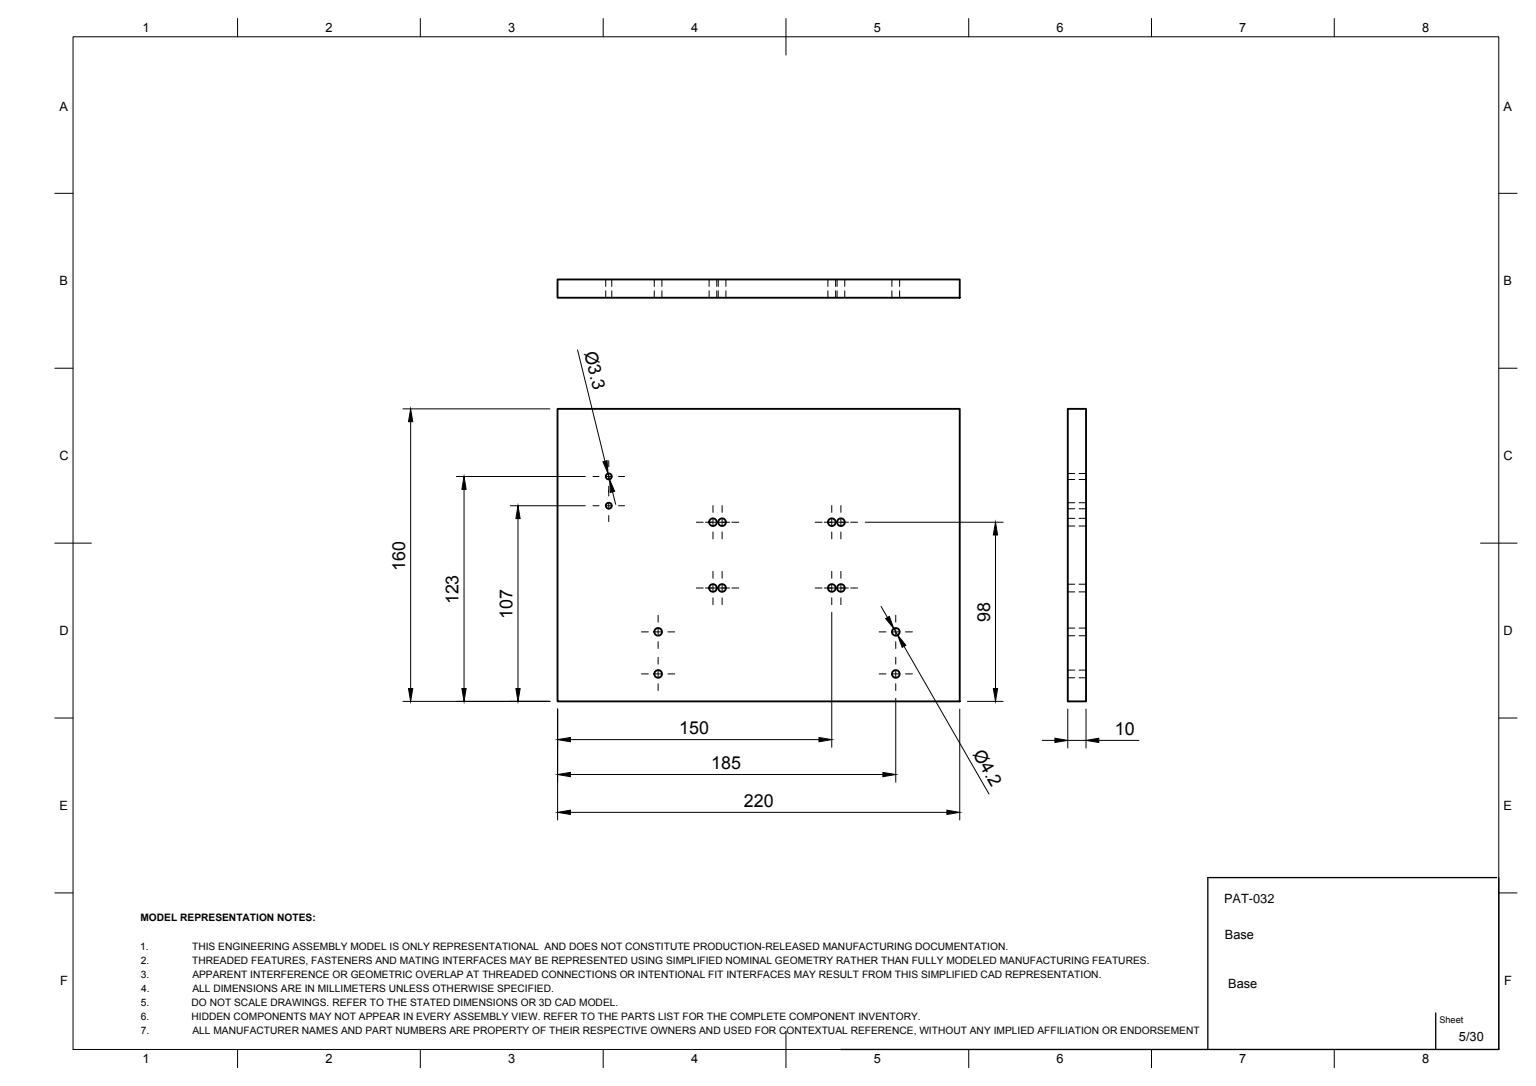
ISO-10303-21;
HEADER;
/* Generated by software containing ST-Developer
 * from STEP Tools, Inc. (www.steptools.com) 
 */

FILE_DESCRIPTION(
/* description */ ('Drill jig with bushing plate'),
/* implementation_level */ '2;1');

FILE_NAME(
/* name */ 'Base.step',
/* time_stamp */ '2026-10-27T10:51:08-07:00',
/* author */ (''),
/* organization */ (''),
/* preprocessor_version */ 'ST-DEVELOPER v20.2',
/* originating_system */ 'Autodesk Translation Framework v15.17.0.0',
/* authorisation */ '');

FILE_SCHEMA (('AUTOMOTIVE_DESIGN { 1 0 10303 214 3 1 1 }'));
ENDSEC;

DATA;
#10=MECHANICAL_DESIGN_GEOMETRIC_PRESENTATION_REPRESENTATION('',(#223),#6638);
#175=SHAPE_REPRESENTATION_RELATIONSHIP('SRR','None',#6739,#199);
#199=ADVANCED_BREP_SHAPE_REPRESENTATION('',(#247),#6612);
#223=STYLED_ITEM('',(#6922),#247);
#247=MANIFOLD_SOLID_BREP('Body1',#3590);
#269=FACE_BOUND('',#734,.T.);
#270=FACE_BOUND('',#735,.T.);
#271=FACE_BOUND('',#736,.T.);
#272=FACE_BOUND('',#737,.T.);
#273=FACE_BOUND('',#738,.T.);
#274=FACE_BOUND('',#739,.T.);
#275=FACE_BOUND('',#740,.T.);
#276=FACE_BOUND('',#741,.T.);
#277=FACE_BOUND('',#742,.T.);
#278=FACE_BOUND('',#743,.T.);
#279=FACE_BOUND('',#744,.T.);
#280=FACE_BOUND('',#745,.T.);
#281=FACE_BOUND('',#746,.T.);
#282=FACE_BOUND('',#747,.T.);
#283=FACE_BOUND('',#749,.T.);
#284=FACE_BOUND('',#750,.T.);
#285=FACE_BOUND('',#751,.T.);
#286=FACE_BOUND('',#752,.T.);
#287=FACE_BOUND('',#753,.T.);
#288=FACE_BOUND('',#754,.T.);
#289=FACE_BOUND('',#755,.T.);
#290=FACE_BOUND('',#756,.T.);
#291=FACE_BOUND('',#757,.T.);
#292=FACE_BOUND('',#758,.T.);
#293=FACE_BOUND('',#759,.T.);
#294=FACE_BOUND('',#760,.T.);
#295=FACE_BOUND('',#761,.T.);
#296=FACE_BOUND('',#762,.T.);
#370=PLANE('',#3926);
#371=PLANE('',#3927);
#372=PLANE('',#3928);
#373=PLANE('',#3929);
#374=PLANE('',#3930);
#375=PLANE('',#3931);
#501=FACE_OUTER_BOUND('',#715,.T.);
#502=FACE_OUTER_BOUND('',#716,.T.);
#503=FACE_OUTER_BOUND('',#717,.T.);
#504=FACE_OUTER_BOUND('',#718,.T.);
#505=FACE_OUTER_BOUND('',#719,.T.);
#506=FACE_OUTER_BOUND('',#720,.T.);
#507=FACE_OUTER_BOUND('',#721,.T.);
#508=FACE_OUTER_BOUND('',#722,.T.);
#509=FACE_OUTER_BOUND('',#723,.T.);
#510=FACE_OUTER_BOUND('',#724,.T.);
#511=FACE_OUTER_BOUND('',#725,.T.);
#512=FACE_OUTER_BOUND('',#726,.T.);
#513=FACE_OUTER_BOUND('',#727,.T.);
#514=FACE_OUTER_BOUND('',#728,.T.);
#515=FACE_OUTER_BOUND('',#729,.T.);
#516=FACE_OUTER_BOUND('',#730,.T.);
#517=FACE_OUTER_BOUND('',#731,.T.);
#518=FACE_OUTER_BOUND('',#732,.T.);
#519=FACE_OUTER_BOUND('',#733,.T.);
#520=FACE_OUTER_BOUND('',#748,.T.);
#715=EDGE_LOOP('',(#2437,#2438,#2439,#2440));
#716=EDGE_LOOP('',(#2441,#2442,#2443,#2444));
#717=EDGE_LOOP('',(#2445,#2446,#2447,#2448));
#718=EDGE_LOOP('',(#2449,#2450,#2451,#2452));
#719=EDGE_LOOP('',(#2453,#2454,#2455,#2456));
#720=EDGE_LOOP('',(#2457,#2458,#2459,#2460));
#721=EDGE_LOOP('',(#2461,#2462,#2463,#2464));
#722=EDGE_LOOP('',(#2465,#2466,#2467,#2468));
#723=EDGE_LOOP('',(#2469,#2470,#2471,#2472));
#724=EDGE_LOOP('',(#2473,#2474,#2475,#2476));
#725=EDGE_LOOP('',(#2477,#2478,#2479,#2480));
#726=EDGE_LOOP('',(#2481,#2482,#2483,#2484));
#727=EDGE_LOOP('',(#2485,#2486,#2487,#2488));
#728=EDGE_LOOP('',(#2489,#2490,#2491,#2492));
#729=EDGE_LOOP('',(#2493,#2494,#2495,#2496));
#730=EDGE_LOOP('',(#2497,#2498,#2499,#2500));
#731=EDGE_LOOP('',(#2501,#2502,#2503,#2504));
#732=EDGE_LOOP('',(#2505,#2506,#2507,#2508));
#733=EDGE_LOOP('',(#2509,#2510,#2511,#2512));
#734=EDGE_LOOP('',(#2513));
#735=EDGE_LOOP('',(#2514));
#736=EDGE_LOOP('',(#2515));
#737=EDGE_LOOP('',(#2516));
#738=EDGE_LOOP('',(#2517));
#739=EDGE_LOOP('',(#2518));
#740=EDGE_LOOP('',(#2519));
#741=EDGE_LOOP('',(#2520));
#742=EDGE_LOOP('',(#2521));
#743=EDGE_LOOP('',(#2522));
#744=EDGE_LOOP('',(#2523));
#745=EDGE_LOOP('',(#2524));
#746=EDGE_LOOP('',(#2525));
#747=EDGE_LOOP('',(#2526));
#748=EDGE_LOOP('',(#2527,#2528,#2529,#2530));
#749=EDGE_LOOP('',(#2531));
#750=EDGE_LOOP('',(#2532));
#751=EDGE_LOOP('',(#2533));
#752=EDGE_LOOP('',(#2534));
#753=EDGE_LOOP('',(#2535));
#754=EDGE_LOOP('',(#2536));
#755=EDGE_LOOP('',(#2537));
#756=EDGE_LOOP('',(#2538));
#757=EDGE_LOOP('',(#2539));
#758=EDGE_LOOP('',(#2540));
#759=EDGE_LOOP('',(#2541));
#760=EDGE_LOOP('',(#2542));
#761=EDGE_LOOP('',(#2543));
#762=EDGE_LOOP('',(#2544));
#1030=LINE('',#5493,#1291);
#1031=LINE('',#5499,#1292);
#1032=LINE('',#5505,#1293);
#1033=LINE('',#5511,#1294);
#1034=LINE('',#5517,#1295);
#1035=LINE('',#5523,#1296);
#1036=LINE('',#5529,#1297);
#1037=LINE('',#5535,#1298);
#1038=LINE('',#5541,#1299);
#1039=LINE('',#5547,#1300);
#1040=LINE('',#5553,#1301);
#1041=LINE('',#5559,#1302);
#1042=LINE('',#5565,#1303);
#1043=LINE('',#5571,#1304);
#1044=LINE('',#5576,#1305);
#1045=LINE('',#5578,#1306);
#1046=LINE('',#5580,#1307);
#1047=LINE('',#5581,#1308);
#1048=LINE('',#5584,#1309);
#1049=LINE('',#5586,#1310);
#1050=LINE('',#5587,#1311);
#1051=LINE('',#5590,#1312);
#1052=LINE('',#5592,#1313);
#1053=LINE('',#5593,#1314);
#1054=LINE('',#5595,#1315);
#1055=LINE('',#5596,#1316);
#1291=VECTOR('',#4339,0.164999999999999);
#1292=VECTOR('',#4346,0.164999999999999);
#1293=VECTOR('',#4353,0.21);
#1294=VECTOR('',#4360,0.21);
#1295=VECTOR('',#4367,0.21);
#1296=VECTOR('',#4374,0.21);
#1297=VECTOR('',#4381,0.21);
#1298=VECTOR('',#4388,0.21);
#1299=VECTOR('',#4395,0.21);
#1300=VECTOR('',#4402,0.21);
#1301=VECTOR('',#4409,0.21);
#1302=VECTOR('',#4416,0.21);
#1303=VECTOR('',#4423,0.21);
#1304=VECTOR('',#4430,0.21);
#1305=VECTOR('',#4435,1.);
#1306=VECTOR('',#4436,1.);
#1307=VECTOR('',#4437,1.);
#1308=VECTOR('',#4438,1.);
#1309=VECTOR('',#4441,1.);
#1310=VECTOR('',#4442,1.);
#1311=VECTOR('',#4443,1.);
#1312=VECTOR('',#4446,1.);
#1313=VECTOR('',#4447,1.);
#1314=VECTOR('',#4448,1.);
#1315=VECTOR('',#4451,1.);
#1316=VECTOR('',#4452,1.);
#1552=CIRCLE('',#3885,0.164999999999999);
#1553=CIRCLE('',#3886,0.164999999999999);
#1554=CIRCLE('',#3888,0.164999999999999);
#1555=CIRCLE('',#3889,0.164999999999999);
#1556=CIRCLE('',#3891,0.21);
#1557=CIRCLE('',#3892,0.21);
#1558=CIRCLE('',#3894,0.21);
#1559=CIRCLE('',#3895,0.21);
#1560=CIRCLE('',#3897,0.21);
#1561=CIRCLE('',#3898,0.21);
#1562=CIRCLE('',#3900,0.21);
#1563=CIRCLE('',#3901,0.21);
#1564=CIRCLE('',#3903,0.21);
#1565=CIRCLE('',#3904,0.21);
#1566=CIRCLE('',#3906,0.21);
#1567=CIRCLE('',#3907,0.21);
#1568=CIRCLE('',#3909,0.21);
#1569=CIRCLE('',#3910,0.21);
#1570=CIRCLE('',#3912,0.21);
#1571=CIRCLE('',#3913,0.21);
#1572=CIRCLE('',#3915,0.21);
#1573=CIRCLE('',#3916,0.21);
#1574=CIRCLE('',#3918,0.21);
#1575=CIRCLE('',#3919,0.21);
#1576=CIRCLE('',#3921,0.21);
#1577=CIRCLE('',#3922,0.21);
#1578=CIRCLE('',#3924,0.21);
#1579=CIRCLE('',#3925,0.21);
#1720=VERTEX_POINT('',#5490);
#1721=VERTEX_POINT('',#5492);
#1722=VERTEX_POINT('',#5496);
#1723=VERTEX_POINT('',#5498);
#1724=VERTEX_POINT('',#5502);
#1725=VERTEX_POINT('',#5504);
#1726=VERTEX_POINT('',#5508);
#1727=VERTEX_POINT('',#5510);
#1728=VERTEX_POINT('',#5514);
#1729=VERTEX_POINT('',#5516);
#1730=VERTEX_POINT('',#5520);
#1731=VERTEX_POINT('',#5522);
#1732=VERTEX_POINT('',#5526);
#1733=VERTEX_POINT('',#5528);
#1734=VERTEX_POINT('',#5532);
#1735=VERTEX_POINT('',#5534);
#1736=VERTEX_POINT('',#5538);
#1737=VERTEX_POINT('',#5540);
#1738=VERTEX_POINT('',#5544);
#1739=VERTEX_POINT('',#5546);
#1740=VERTEX_POINT('',#5550);
#1741=VERTEX_POINT('',#5552);
#1742=VERTEX_POINT('',#5556);
#1743=VERTEX_POINT('',#5558);
#1744=VERTEX_POINT('',#5562);
#1745=VERTEX_POINT('',#5564);
#1746=VERTEX_POINT('',#5568);
#1747=VERTEX_POINT('',#5570);
#1748=VERTEX_POINT('',#5574);
#1749=VERTEX_POINT('',#5575);
#1750=VERTEX_POINT('',#5577);
#1751=VERTEX_POINT('',#5579);
#1752=VERTEX_POINT('',#5583);
#1753=VERTEX_POINT('',#5585);
#1754=VERTEX_POINT('',#5589);
#1755=VERTEX_POINT('',#5591);
#2006=EDGE_CURVE('',#1720,#1720,#1552,.T.);
#2007=EDGE_CURVE('',#1720,#1721,#1030,.T.);
#2008=EDGE_CURVE('',#1721,#1721,#1553,.T.);
#2009=EDGE_CURVE('',#1722,#1722,#1554,.T.);
#2010=EDGE_CURVE('',#1722,#1723,#1031,.T.);
#2011=EDGE_CURVE('',#1723,#1723,#1555,.T.);
#2012=EDGE_CURVE('',#1724,#1724,#1556,.T.);
#2013=EDGE_CURVE('',#1724,#1725,#1032,.T.);
#2014=EDGE_CURVE('',#1725,#1725,#1557,.T.);
#2015=EDGE_CURVE('',#1726,#1726,#1558,.T.);
#2016=EDGE_CURVE('',#1726,#1727,#1033,.T.);
#2017=EDGE_CURVE('',#1727,#1727,#1559,.T.);
#2018=EDGE_CURVE('',#1728,#1728,#1560,.T.);
#2019=EDGE_CURVE('',#1728,#1729,#1034,.T.);
#2020=EDGE_CURVE('',#1729,#1729,#1561,.T.);
#2021=EDGE_CURVE('',#1730,#1730,#1562,.T.);
#2022=EDGE_CURVE('',#1730,#1731,#1035,.T.);
#2023=EDGE_CURVE('',#1731,#1731,#1563,.T.);
#2024=EDGE_CURVE('',#1732,#1732,#1564,.T.);
#2025=EDGE_CURVE('',#1732,#1733,#1036,.T.);
#2026=EDGE_CURVE('',#1733,#1733,#1565,.T.);
#2027=EDGE_CURVE('',#1734,#1734,#1566,.T.);
#2028=EDGE_CURVE('',#1734,#1735,#1037,.T.);
#2029=EDGE_CURVE('',#1735,#1735,#1567,.T.);
#2030=EDGE_CURVE('',#1736,#1736,#1568,.T.);
#2031=EDGE_CURVE('',#1736,#1737,#1038,.T.);
#2032=EDGE_CURVE('',#1737,#1737,#1569,.T.);
#2033=EDGE_CURVE('',#1738,#1738,#1570,.T.);
#2034=EDGE_CURVE('',#1738,#1739,#1039,.T.);
#2035=EDGE_CURVE('',#1739,#1739,#1571,.T.);
#2036=EDGE_CURVE('',#1740,#1740,#1572,.T.);
#2037=EDGE_CURVE('',#1740,#1741,#1040,.T.);
#2038=EDGE_CURVE('',#1741,#1741,#1573,.T.);
#2039=EDGE_CURVE('',#1742,#1742,#1574,.T.);
#2040=EDGE_CURVE('',#1742,#1743,#1041,.T.);
#2041=EDGE_CURVE('',#1743,#1743,#1575,.T.);
#2042=EDGE_CURVE('',#1744,#1744,#1576,.T.);
#2043=EDGE_CURVE('',#1744,#1745,#1042,.T.);
#2044=EDGE_CURVE('',#1745,#1745,#1577,.T.);
#2045=EDGE_CURVE('',#1746,#1746,#1578,.T.);
#2046=EDGE_CURVE('',#1746,#1747,#1043,.T.);
#2047=EDGE_CURVE('',#1747,#1747,#1579,.T.);
#2048=EDGE_CURVE('',#1748,#1749,#1044,.T.);
#2049=EDGE_CURVE('',#1749,#1750,#1045,.T.);
#2050=EDGE_CURVE('',#1751,#1750,#1046,.T.);
#2051=EDGE_CURVE('',#1748,#1751,#1047,.T.);
#2052=EDGE_CURVE('',#1752,#1748,#1048,.T.);
#2053=EDGE_CURVE('',#1753,#1751,#1049,.T.);
#2054=EDGE_CURVE('',#1752,#1753,#1050,.T.);
#2055=EDGE_CURVE('',#1754,#1752,#1051,.T.);
#2056=EDGE_CURVE('',#1755,#1753,#1052,.T.);
#2057=EDGE_CURVE('',#1754,#1755,#1053,.T.);
#2058=EDGE_CURVE('',#1749,#1754,#1054,.T.);
#2059=EDGE_CURVE('',#1750,#1755,#1055,.T.);
#2437=ORIENTED_EDGE('',*,*,#2006,.F.);
#2438=ORIENTED_EDGE('',*,*,#2007,.T.);
#2439=ORIENTED_EDGE('',*,*,#2008,.F.);
#2440=ORIENTED_EDGE('',*,*,#2007,.F.);
#2441=ORIENTED_EDGE('',*,*,#2009,.F.);
#2442=ORIENTED_EDGE('',*,*,#2010,.T.);
#2443=ORIENTED_EDGE('',*,*,#2011,.F.);
#2444=ORIENTED_EDGE('',*,*,#2010,.F.);
#2445=ORIENTED_EDGE('',*,*,#2012,.F.);
#2446=ORIENTED_EDGE('',*,*,#2013,.T.);
#2447=ORIENTED_EDGE('',*,*,#2014,.F.);
#2448=ORIENTED_EDGE('',*,*,#2013,.F.);
#2449=ORIENTED_EDGE('',*,*,#2015,.F.);
#2450=ORIENTED_EDGE('',*,*,#2016,.T.);
#2451=ORIENTED_EDGE('',*,*,#2017,.F.);
#2452=ORIENTED_EDGE('',*,*,#2016,.F.);
#2453=ORIENTED_EDGE('',*,*,#2018,.F.);
#2454=ORIENTED_EDGE('',*,*,#2019,.T.);
#2455=ORIENTED_EDGE('',*,*,#2020,.F.);
#2456=ORIENTED_EDGE('',*,*,#2019,.F.);
#2457=ORIENTED_EDGE('',*,*,#2021,.F.);
#2458=ORIENTED_EDGE('',*,*,#2022,.T.);
#2459=ORIENTED_EDGE('',*,*,#2023,.F.);
#2460=ORIENTED_EDGE('',*,*,#2022,.F.);
#2461=ORIENTED_EDGE('',*,*,#2024,.F.);
#2462=ORIENTED_EDGE('',*,*,#2025,.T.);
#2463=ORIENTED_EDGE('',*,*,#2026,.F.);
#2464=ORIENTED_EDGE('',*,*,#2025,.F.);
#2465=ORIENTED_EDGE('',*,*,#2027,.F.);
#2466=ORIENTED_EDGE('',*,*,#2028,.T.);
#2467=ORIENTED_EDGE('',*,*,#2029,.F.);
#2468=ORIENTED_EDGE('',*,*,#2028,.F.);
#2469=ORIENTED_EDGE('',*,*,#2030,.F.);
#2470=ORIENTED_EDGE('',*,*,#2031,.T.);
#2471=ORIENTED_EDGE('',*,*,#2032,.F.);
#2472=ORIENTED_EDGE('',*,*,#2031,.F.);
#2473=ORIENTED_EDGE('',*,*,#2033,.F.);
#2474=ORIENTED_EDGE('',*,*,#2034,.T.);
#2475=ORIENTED_EDGE('',*,*,#2035,.F.);
#2476=ORIENTED_EDGE('',*,*,#2034,.F.);
#2477=ORIENTED_EDGE('',*,*,#2036,.F.);
#2478=ORIENTED_EDGE('',*,*,#2037,.T.);
#2479=ORIENTED_EDGE('',*,*,#2038,.F.);
#2480=ORIENTED_EDGE('',*,*,#2037,.F.);
#2481=ORIENTED_EDGE('',*,*,#2039,.F.);
#2482=ORIENTED_EDGE('',*,*,#2040,.T.);
#2483=ORIENTED_EDGE('',*,*,#2041,.F.);
#2484=ORIENTED_EDGE('',*,*,#2040,.F.);
#2485=ORIENTED_EDGE('',*,*,#2042,.F.);
#2486=ORIENTED_EDGE('',*,*,#2043,.T.);
#2487=ORIENTED_EDGE('',*,*,#2044,.F.);
#2488=ORIENTED_EDGE('',*,*,#2043,.F.);
#2489=ORIENTED_EDGE('',*,*,#2045,.F.);
#2490=ORIENTED_EDGE('',*,*,#2046,.T.);
#2491=ORIENTED_EDGE('',*,*,#2047,.F.);
#2492=ORIENTED_EDGE('',*,*,#2046,.F.);
#2493=ORIENTED_EDGE('',*,*,#2048,.T.);
#2494=ORIENTED_EDGE('',*,*,#2049,.T.);
#2495=ORIENTED_EDGE('',*,*,#2050,.F.);
#2496=ORIENTED_EDGE('',*,*,#2051,.F.);
#2497=ORIENTED_EDGE('',*,*,#2052,.T.);
#2498=ORIENTED_EDGE('',*,*,#2051,.T.);
#2499=ORIENTED_EDGE('',*,*,#2053,.F.);
#2500=ORIENTED_EDGE('',*,*,#2054,.F.);
#2501=ORIENTED_EDGE('',*,*,#2055,.T.);
#2502=ORIENTED_EDGE('',*,*,#2054,.T.);
#2503=ORIENTED_EDGE('',*,*,#2056,.F.);
#2504=ORIENTED_EDGE('',*,*,#2057,.F.);
#2505=ORIENTED_EDGE('',*,*,#2058,.T.);
#2506=ORIENTED_EDGE('',*,*,#2057,.T.);
#2507=ORIENTED_EDGE('',*,*,#2059,.F.);
#2508=ORIENTED_EDGE('',*,*,#2049,.F.);
#2509=ORIENTED_EDGE('',*,*,#2059,.T.);
#2510=ORIENTED_EDGE('',*,*,#2056,.T.);
#2511=ORIENTED_EDGE('',*,*,#2053,.T.);
#2512=ORIENTED_EDGE('',*,*,#2050,.T.);
#2513=ORIENTED_EDGE('',*,*,#2014,.T.);
#2514=ORIENTED_EDGE('',*,*,#2017,.T.);
#2515=ORIENTED_EDGE('',*,*,#2020,.T.);
#2516=ORIENTED_EDGE('',*,*,#2023,.T.);
#2517=ORIENTED_EDGE('',*,*,#2047,.T.);
#2518=ORIENTED_EDGE('',*,*,#2044,.T.);
#2519=ORIENTED_EDGE('',*,*,#2041,.T.);
#2520=ORIENTED_EDGE('',*,*,#2038,.T.);
#2521=ORIENTED_EDGE('',*,*,#2035,.T.);
#2522=ORIENTED_EDGE('',*,*,#2032,.T.);
#2523=ORIENTED_EDGE('',*,*,#2029,.T.);
#2524=ORIENTED_EDGE('',*,*,#2026,.T.);
#2525=ORIENTED_EDGE('',*,*,#2011,.T.);
#2526=ORIENTED_EDGE('',*,*,#2008,.T.);
#2527=ORIENTED_EDGE('',*,*,#2058,.F.);
#2528=ORIENTED_EDGE('',*,*,#2048,.F.);
#2529=ORIENTED_EDGE('',*,*,#2052,.F.);
#2530=ORIENTED_EDGE('',*,*,#2055,.F.);
#2531=ORIENTED_EDGE('',*,*,#2012,.T.);
#2532=ORIENTED_EDGE('',*,*,#2015,.T.);
#2533=ORIENTED_EDGE('',*,*,#2018,.T.);
#2534=ORIENTED_EDGE('',*,*,#2021,.T.);
#2535=ORIENTED_EDGE('',*,*,#2045,.T.);
#2536=ORIENTED_EDGE('',*,*,#2042,.T.);
#2537=ORIENTED_EDGE('',*,*,#2039,.T.);
#2538=ORIENTED_EDGE('',*,*,#2036,.T.);
#2539=ORIENTED_EDGE('',*,*,#2033,.T.);
#2540=ORIENTED_EDGE('',*,*,#2030,.T.);
#2541=ORIENTED_EDGE('',*,*,#2027,.T.);
#2542=ORIENTED_EDGE('',*,*,#2024,.T.);
#2543=ORIENTED_EDGE('',*,*,#2009,.T.);
#2544=ORIENTED_EDGE('',*,*,#2006,.T.);
#3299=CYLINDRICAL_SURFACE('',#3884,0.164999999999999);
#3300=CYLINDRICAL_SURFACE('',#3887,0.164999999999999);
#3301=CYLINDRICAL_SURFACE('',#3890,0.21);
#3302=CYLINDRICAL_SURFACE('',#3893,0.21);
#3303=CYLINDRICAL_SURFACE('',#3896,0.21);
#3304=CYLINDRICAL_SURFACE('',#3899,0.21);
#3305=CYLINDRICAL_SURFACE('',#3902,0.21);
#3306=CYLINDRICAL_SURFACE('',#3905,0.21);
#3307=CYLINDRICAL_SURFACE('',#3908,0.21);
#3308=CYLINDRICAL_SURFACE('',#3911,0.21);
#3309=CYLINDRICAL_SURFACE('',#3914,0.21);
#3310=CYLINDRICAL_SURFACE('',#3917,0.21);
#3311=CYLINDRICAL_SURFACE('',#3920,0.21);
#3312=CYLINDRICAL_SURFACE('',#3923,0.21);
#3376=ADVANCED_FACE('',(#501),#3299,.F.);
#3377=ADVANCED_FACE('',(#502),#3300,.F.);
#3378=ADVANCED_FACE('',(#503),#3301,.F.);
#3379=ADVANCED_FACE('',(#504),#3302,.F.);
#3380=ADVANCED_FACE('',(#505),#3303,.F.);
#3381=ADVANCED_FACE('',(#506),#3304,.F.);
#3382=ADVANCED_FACE('',(#507),#3305,.F.);
#3383=ADVANCED_FACE('',(#508),#3306,.F.);
#3384=ADVANCED_FACE('',(#509),#3307,.F.);
#3385=ADVANCED_FACE('',(#510),#3308,.F.);
#3386=ADVANCED_FACE('',(#511),#3309,.F.);
#3387=ADVANCED_FACE('',(#512),#3310,.F.);
#3388=ADVANCED_FACE('',(#513),#3311,.F.);
#3389=ADVANCED_FACE('',(#514),#3312,.F.);
#3390=ADVANCED_FACE('',(#515),#370,.T.);
#3391=ADVANCED_FACE('',(#516),#371,.T.);
#3392=ADVANCED_FACE('',(#517),#372,.T.);
#3393=ADVANCED_FACE('',(#518),#373,.T.);
#3394=ADVANCED_FACE('',(#519,#269,#270,#271,#272,#273,#274,#275,#276,#277,
#278,#279,#280,#281,#282),#374,.T.);
#3395=ADVANCED_FACE('',(#520,#283,#284,#285,#286,#287,#288,#289,#290,#291,
#292,#293,#294,#295,#296),#375,.F.);
#3590=CLOSED_SHELL('',(#3376,#3377,#3378,#3379,#3380,#3381,#3382,#3383,
#3384,#3385,#3386,#3387,#3388,#3389,#3390,#3391,#3392,#3393,#3394,#3395));
#3883=AXIS2_PLACEMENT_3D('',#5488,#4333,#4334);
#3884=AXIS2_PLACEMENT_3D('',#5489,#4335,#4336);
#3885=AXIS2_PLACEMENT_3D('',#5491,#4337,#4338);
#3886=AXIS2_PLACEMENT_3D('',#5494,#4340,#4341);
#3887=AXIS2_PLACEMENT_3D('',#5495,#4342,#4343);
#3888=AXIS2_PLACEMENT_3D('',#5497,#4344,#4345);
#3889=AXIS2_PLACEMENT_3D('',#5500,#4347,#4348);
#3890=AXIS2_PLACEMENT_3D('',#5501,#4349,#4350);
#3891=AXIS2_PLACEMENT_3D('',#5503,#4351,#4352);
#3892=AXIS2_PLACEMENT_3D('',#5506,#4354,#4355);
#3893=AXIS2_PLACEMENT_3D('',#5507,#4356,#4357);
#3894=AXIS2_PLACEMENT_3D('',#5509,#4358,#4359);
#3895=AXIS2_PLACEMENT_3D('',#5512,#4361,#4362);
#3896=AXIS2_PLACEMENT_3D('',#5513,#4363,#4364);
#3897=AXIS2_PLACEMENT_3D('',#5515,#4365,#4366);
#3898=AXIS2_PLACEMENT_3D('',#5518,#4368,#4369);
#3899=AXIS2_PLACEMENT_3D('',#5519,#4370,#4371);
#3900=AXIS2_PLACEMENT_3D('',#5521,#4372,#4373);
#3901=AXIS2_PLACEMENT_3D('',#5524,#4375,#4376);
#3902=AXIS2_PLACEMENT_3D('',#5525,#4377,#4378);
#3903=AXIS2_PLACEMENT_3D('',#5527,#4379,#4380);
#3904=AXIS2_PLACEMENT_3D('',#5530,#4382,#4383);
#3905=AXIS2_PLACEMENT_3D('',#5531,#4384,#4385);
#3906=AXIS2_PLACEMENT_3D('',#5533,#4386,#4387);
#3907=AXIS2_PLACEMENT_3D('',#5536,#4389,#4390);
#3908=AXIS2_PLACEMENT_3D('',#5537,#4391,#4392);
#3909=AXIS2_PLACEMENT_3D('',#5539,#4393,#4394);
#3910=AXIS2_PLACEMENT_3D('',#5542,#4396,#4397);
#3911=AXIS2_PLACEMENT_3D('',#5543,#4398,#4399);
#3912=AXIS2_PLACEMENT_3D('',#5545,#4400,#4401);
#3913=AXIS2_PLACEMENT_3D('',#5548,#4403,#4404);
#3914=AXIS2_PLACEMENT_3D('',#5549,#4405,#4406);
#3915=AXIS2_PLACEMENT_3D('',#5551,#4407,#4408);
#3916=AXIS2_PLACEMENT_3D('',#5554,#4410,#4411);
#3917=AXIS2_PLACEMENT_3D('',#5555,#4412,#4413);
#3918=AXIS2_PLACEMENT_3D('',#5557,#4414,#4415);
#3919=AXIS2_PLACEMENT_3D('',#5560,#4417,#4418);
#3920=AXIS2_PLACEMENT_3D('',#5561,#4419,#4420);
#3921=AXIS2_PLACEMENT_3D('',#5563,#4421,#4422);
#3922=AXIS2_PLACEMENT_3D('',#5566,#4424,#4425);
#3923=AXIS2_PLACEMENT_3D('',#5567,#4426,#4427);
#3924=AXIS2_PLACEMENT_3D('',#5569,#4428,#4429);
#3925=AXIS2_PLACEMENT_3D('',#5572,#4431,#4432);
#3926=AXIS2_PLACEMENT_3D('',#5573,#4433,#4434);
#3927=AXIS2_PLACEMENT_3D('',#5582,#4439,#4440);
#3928=AXIS2_PLACEMENT_3D('',#5588,#4444,#4445);
#3929=AXIS2_PLACEMENT_3D('',#5594,#4449,#4450);
#3930=AXIS2_PLACEMENT_3D('',#5597,#4453,#4454);
#3931=AXIS2_PLACEMENT_3D('',#5598,#4455,#4456);
#4333=DIRECTION('axis',(0.,0.,1.));
#4334=DIRECTION('refdir',(1.,0.,0.));
#4335=DIRECTION('center_axis',(0.,0.,1.));
#4336=DIRECTION('ref_axis',(1.,0.,0.));
#4337=DIRECTION('center_axis',(0.,0.,1.));
#4338=DIRECTION('ref_axis',(1.,0.,0.));
#4339=DIRECTION('',(0.,0.,1.));
#4340=DIRECTION('center_axis',(0.,0.,-1.));
#4341=DIRECTION('ref_axis',(1.,0.,0.));
#4342=DIRECTION('center_axis',(0.,0.,1.));
#4343=DIRECTION('ref_axis',(1.,0.,0.));
#4344=DIRECTION('center_axis',(0.,0.,1.));
#4345=DIRECTION('ref_axis',(1.,0.,0.));
#4346=DIRECTION('',(0.,0.,1.));
#4347=DIRECTION('center_axis',(0.,0.,-1.));
#4348=DIRECTION('ref_axis',(1.,0.,0.));
#4349=DIRECTION('center_axis',(0.,0.,1.));
#4350=DIRECTION('ref_axis',(1.,0.,0.));
#4351=DIRECTION('center_axis',(0.,0.,1.));
#4352=DIRECTION('ref_axis',(1.,0.,0.));
#4353=DIRECTION('',(0.,0.,1.));
#4354=DIRECTION('center_axis',(0.,0.,-1.));
#4355=DIRECTION('ref_axis',(1.,0.,0.));
#4356=DIRECTION('center_axis',(0.,0.,1.));
#4357=DIRECTION('ref_axis',(1.,0.,0.));
#4358=DIRECTION('center_axis',(0.,0.,1.));
#4359=DIRECTION('ref_axis',(1.,0.,0.));
#4360=DIRECTION('',(0.,0.,1.));
#4361=DIRECTION('center_axis',(0.,0.,-1.));
#4362=DIRECTION('ref_axis',(1.,0.,0.));
#4363=DIRECTION('center_axis',(0.,0.,1.));
#4364=DIRECTION('ref_axis',(1.,0.,0.));
#4365=DIRECTION('center_axis',(0.,0.,1.));
#4366=DIRECTION('ref_axis',(1.,0.,0.));
#4367=DIRECTION('',(0.,0.,1.));
#4368=DIRECTION('center_axis',(0.,0.,-1.));
#4369=DIRECTION('ref_axis',(1.,0.,0.));
#4370=DIRECTION('center_axis',(0.,0.,1.));
#4371=DIRECTION('ref_axis',(1.,0.,0.));
#4372=DIRECTION('center_axis',(0.,0.,1.));
#4373=DIRECTION('ref_axis',(1.,0.,0.));
#4374=DIRECTION('',(0.,0.,1.));
#4375=DIRECTION('center_axis',(0.,0.,-1.));
#4376=DIRECTION('ref_axis',(1.,0.,0.));
#4377=DIRECTION('center_axis',(0.,0.,1.));
#4378=DIRECTION('ref_axis',(1.,0.,0.));
#4379=DIRECTION('center_axis',(0.,0.,1.));
#4380=DIRECTION('ref_axis',(1.,0.,0.));
#4381=DIRECTION('',(0.,0.,1.));
#4382=DIRECTION('center_axis',(0.,0.,-1.));
#4383=DIRECTION('ref_axis',(1.,0.,0.));
#4384=DIRECTION('center_axis',(0.,0.,1.));
#4385=DIRECTION('ref_axis',(1.,0.,0.));
#4386=DIRECTION('center_axis',(0.,0.,1.));
#4387=DIRECTION('ref_axis',(1.,0.,0.));
#4388=DIRECTION('',(0.,0.,1.));
#4389=DIRECTION('center_axis',(0.,0.,-1.));
#4390=DIRECTION('ref_axis',(1.,0.,0.));
#4391=DIRECTION('center_axis',(0.,0.,1.));
#4392=DIRECTION('ref_axis',(1.,0.,0.));
#4393=DIRECTION('center_axis',(0.,0.,1.));
#4394=DIRECTION('ref_axis',(1.,0.,0.));
#4395=DIRECTION('',(0.,0.,1.));
#4396=DIRECTION('center_axis',(0.,0.,-1.));
#4397=DIRECTION('ref_axis',(1.,0.,0.));
#4398=DIRECTION('center_axis',(0.,0.,1.));
#4399=DIRECTION('ref_axis',(1.,0.,0.));
#4400=DIRECTION('center_axis',(0.,0.,1.));
#4401=DIRECTION('ref_axis',(1.,0.,0.));
#4402=DIRECTION('',(0.,0.,1.));
#4403=DIRECTION('center_axis',(0.,0.,-1.));
#4404=DIRECTION('ref_axis',(1.,0.,0.));
#4405=DIRECTION('center_axis',(0.,0.,1.));
#4406=DIRECTION('ref_axis',(1.,0.,0.));
#4407=DIRECTION('center_axis',(0.,0.,1.));
#4408=DIRECTION('ref_axis',(1.,0.,0.));
#4409=DIRECTION('',(0.,0.,1.));
#4410=DIRECTION('center_axis',(0.,0.,-1.));
#4411=DIRECTION('ref_axis',(1.,0.,0.));
#4412=DIRECTION('center_axis',(0.,0.,1.));
#4413=DIRECTION('ref_axis',(1.,0.,0.));
#4414=DIRECTION('center_axis',(0.,0.,1.));
#4415=DIRECTION('ref_axis',(1.,0.,0.));
#4416=DIRECTION('',(0.,0.,1.));
#4417=DIRECTION('center_axis',(0.,0.,-1.));
#4418=DIRECTION('ref_axis',(1.,0.,0.));
#4419=DIRECTION('center_axis',(0.,0.,1.));
#4420=DIRECTION('ref_axis',(1.,0.,0.));
#4421=DIRECTION('center_axis',(0.,0.,1.));
#4422=DIRECTION('ref_axis',(1.,0.,0.));
#4423=DIRECTION('',(0.,0.,1.));
#4424=DIRECTION('center_axis',(0.,0.,-1.));
#4425=DIRECTION('ref_axis',(1.,0.,0.));
#4426=DIRECTION('center_axis',(0.,0.,1.));
#4427=DIRECTION('ref_axis',(1.,0.,0.));
#4428=DIRECTION('center_axis',(0.,0.,1.));
#4429=DIRECTION('ref_axis',(1.,0.,0.));
#4430=DIRECTION('',(0.,0.,1.));
#4431=DIRECTION('center_axis',(0.,0.,-1.));
#4432=DIRECTION('ref_axis',(1.,0.,0.));
#4433=DIRECTION('center_axis',(0.,1.,0.));
#4434=DIRECTION('ref_axis',(-1.,0.,0.));
#4435=DIRECTION('',(-1.,0.,0.));
#4436=DIRECTION('',(0.,0.,1.));
#4437=DIRECTION('',(-1.,0.,0.));
#4438=DIRECTION('',(0.,0.,1.));
#4439=DIRECTION('center_axis',(1.,0.,0.));
#4440=DIRECTION('ref_axis',(0.,1.,0.));
#4441=DIRECTION('',(0.,1.,0.));
#4442=DIRECTION('',(0.,1.,0.));
#4443=DIRECTION('',(0.,0.,1.));
#4444=DIRECTION('center_axis',(0.,-1.,0.));
#4445=DIRECTION('ref_axis',(1.,0.,0.));
#4446=DIRECTION('',(1.,0.,0.));
#4447=DIRECTION('',(1.,0.,0.));
#4448=DIRECTION('',(0.,0.,1.));
#4449=DIRECTION('center_axis',(-1.,0.,0.));
#4450=DIRECTION('ref_axis',(0.,-1.,0.));
#4451=DIRECTION('',(0.,-1.,0.));
#4452=DIRECTION('',(0.,-1.,0.));
#4453=DIRECTION('center_axis',(0.,0.,1.));
#4454=DIRECTION('ref_axis',(1.,0.,0.));
#4455=DIRECTION('center_axis',(0.,0.,1.));
#4456=DIRECTION('ref_axis',(1.,0.,0.));
#5488=CARTESIAN_POINT('',(0.,0.,0.));
#5489=CARTESIAN_POINT('Origin',(9.2,2.7,-0.1));
#5490=CARTESIAN_POINT('',(9.035,2.7,0.));
#5491=CARTESIAN_POINT('Origin',(9.2,2.7,0.));
#5492=CARTESIAN_POINT('',(9.035,2.7,1.));
#5493=CARTESIAN_POINT('',(9.035,2.7,-0.1));
#5494=CARTESIAN_POINT('Origin',(9.2,2.7,1.));
#5495=CARTESIAN_POINT('Origin',(9.2,4.3,-0.1));
#5496=CARTESIAN_POINT('',(9.035,4.3,0.));
#5497=CARTESIAN_POINT('Origin',(9.2,4.3,0.));
#5498=CARTESIAN_POINT('',(9.035,4.3,1.));
#5499=CARTESIAN_POINT('',(9.035,4.3,-0.1));
#5500=CARTESIAN_POINT('Origin',(9.2,4.3,1.));
#5501=CARTESIAN_POINT('Origin',(3.5,-1.8,-0.1));
#5502=CARTESIAN_POINT('',(3.29,-1.8,0.));
#5503=CARTESIAN_POINT('Origin',(3.5,-1.8,0.));
#5504=CARTESIAN_POINT('',(3.29,-1.8,1.));
#5505=CARTESIAN_POINT('',(3.29,-1.8,-0.1));
#5506=CARTESIAN_POINT('Origin',(3.5,-1.8,1.));
#5507=CARTESIAN_POINT('Origin',(-3.5,1.8,-0.1));
#5508=CARTESIAN_POINT('',(-3.71,1.8,0.));
#5509=CARTESIAN_POINT('Origin',(-3.5,1.8,0.));
#5510=CARTESIAN_POINT('',(-3.71,1.8,1.));
#5511=CARTESIAN_POINT('',(-3.71,1.8,-0.1));
#5512=CARTESIAN_POINT('Origin',(-3.5,1.8,1.));
#5513=CARTESIAN_POINT('Origin',(-3.5,-1.8,-0.1));
#5514=CARTESIAN_POINT('',(-3.71,-1.8,0.));
#5515=CARTESIAN_POINT('Origin',(-3.5,-1.8,0.));
#5516=CARTESIAN_POINT('',(-3.71,-1.8,1.));
#5517=CARTESIAN_POINT('',(-3.71,-1.8,-0.1));
#5518=CARTESIAN_POINT('Origin',(-3.5,-1.8,1.));
#5519=CARTESIAN_POINT('Origin',(3.5,1.8,-0.1));
#5520=CARTESIAN_POINT('',(3.29,1.8,0.));
#5521=CARTESIAN_POINT('Origin',(3.5,1.8,0.));
#5522=CARTESIAN_POINT('',(3.29,1.8,1.));
#5523=CARTESIAN_POINT('',(3.29,1.8,-0.1));
#5524=CARTESIAN_POINT('Origin',(3.5,1.8,1.));
#5525=CARTESIAN_POINT('Origin',(3.,-1.8,-0.1));
#5526=CARTESIAN_POINT('',(2.79,-1.8,0.));
#5527=CARTESIAN_POINT('Origin',(3.,-1.8,0.));
#5528=CARTESIAN_POINT('',(2.79,-1.8,1.));
#5529=CARTESIAN_POINT('',(2.79,-1.8,-0.1));
#5530=CARTESIAN_POINT('Origin',(3.,-1.8,1.));
#5531=CARTESIAN_POINT('Origin',(-3.,1.8,-0.1));
#5532=CARTESIAN_POINT('',(-3.21,1.8,0.));
#5533=CARTESIAN_POINT('Origin',(-3.,1.8,0.));
#5534=CARTESIAN_POINT('',(-3.21,1.8,1.));
#5535=CARTESIAN_POINT('',(-3.21,1.8,-0.1));
#5536=CARTESIAN_POINT('Origin',(-3.,1.8,1.));
#5537=CARTESIAN_POINT('Origin',(-3.,-1.8,-0.1));
#5538=CARTESIAN_POINT('',(-3.21,-1.8,0.));
#5539=CARTESIAN_POINT('Origin',(-3.,-1.8,0.));
#5540=CARTESIAN_POINT('',(-3.21,-1.8,1.));
#5541=CARTESIAN_POINT('',(-3.21,-1.8,-0.1));
#5542=CARTESIAN_POINT('Origin',(-3.,-1.8,1.));
#5543=CARTESIAN_POINT('Origin',(3.,1.8,-0.1));
#5544=CARTESIAN_POINT('',(2.79,1.8,0.));
#5545=CARTESIAN_POINT('Origin',(3.,1.8,0.));
#5546=CARTESIAN_POINT('',(2.79,1.8,1.));
#5547=CARTESIAN_POINT('',(2.79,1.8,-0.1));
#5548=CARTESIAN_POINT('Origin',(3.,1.8,1.));
#5549=CARTESIAN_POINT('Origin',(6.5,-6.5,-0.1));
#5550=CARTESIAN_POINT('',(6.29,-6.5,0.));
#5551=CARTESIAN_POINT('Origin',(6.5,-6.5,0.));
#5552=CARTESIAN_POINT('',(6.29,-6.5,1.));
#5553=CARTESIAN_POINT('',(6.29,-6.5,-0.1));
#5554=CARTESIAN_POINT('Origin',(6.5,-6.5,1.));
#5555=CARTESIAN_POINT('Origin',(-6.5,-4.2,-0.1));
#5556=CARTESIAN_POINT('',(-6.71,-4.2,0.));
#5557=CARTESIAN_POINT('Origin',(-6.5,-4.2,0.));
#5558=CARTESIAN_POINT('',(-6.71,-4.2,1.));
#5559=CARTESIAN_POINT('',(-6.71,-4.2,-0.1));
#5560=CARTESIAN_POINT('Origin',(-6.5,-4.2,1.));
#5561=CARTESIAN_POINT('Origin',(-6.5,-6.5,-0.1));
#5562=CARTESIAN_POINT('',(-6.71,-6.5,0.));
#5563=CARTESIAN_POINT('Origin',(-6.5,-6.5,0.));
#5564=CARTESIAN_POINT('',(-6.71,-6.5,1.));
#5565=CARTESIAN_POINT('',(-6.71,-6.5,-0.1));
#5566=CARTESIAN_POINT('Origin',(-6.5,-6.5,1.));
#5567=CARTESIAN_POINT('Origin',(6.5,-4.2,-0.1));
#5568=CARTESIAN_POINT('',(6.29,-4.2,0.));
#5569=CARTESIAN_POINT('Origin',(6.5,-4.2,0.));
#5570=CARTESIAN_POINT('',(6.29,-4.2,1.));
#5571=CARTESIAN_POINT('',(6.29,-4.2,-0.1));
#5572=CARTESIAN_POINT('Origin',(6.5,-4.2,1.));
#5573=CARTESIAN_POINT('Origin',(12.,8.,0.));
#5574=CARTESIAN_POINT('',(12.,8.,0.));
#5575=CARTESIAN_POINT('',(-10.,8.,0.));
#5576=CARTESIAN_POINT('',(12.,8.,0.));
#5577=CARTESIAN_POINT('',(-10.,8.,1.));
#5578=CARTESIAN_POINT('',(-10.,8.,0.));
#5579=CARTESIAN_POINT('',(12.,8.,1.));
#5580=CARTESIAN_POINT('',(12.,8.,1.));
#5581=CARTESIAN_POINT('',(12.,8.,0.));
#5582=CARTESIAN_POINT('Origin',(12.,-8.,0.));
#5583=CARTESIAN_POINT('',(12.,-8.,0.));
#5584=CARTESIAN_POINT('',(12.,-8.,0.));
#5585=CARTESIAN_POINT('',(12.,-8.,1.));
#5586=CARTESIAN_POINT('',(12.,-8.,1.));
#5587=CARTESIAN_POINT('',(12.,-8.,0.));
#5588=CARTESIAN_POINT('Origin',(-10.,-8.,0.));
#5589=CARTESIAN_POINT('',(-10.,-8.,0.));
#5590=CARTESIAN_POINT('',(-10.,-8.,0.));
#5591=CARTESIAN_POINT('',(-10.,-8.,1.));
#5592=CARTESIAN_POINT('',(-10.,-8.,1.));
#5593=CARTESIAN_POINT('',(-10.,-8.,0.));
#5594=CARTESIAN_POINT('Origin',(-10.,8.,0.));
#5595=CARTESIAN_POINT('',(-10.,8.,0.));
#5596=CARTESIAN_POINT('',(-10.,8.,1.));
#5597=CARTESIAN_POINT('Origin',(1.,0.,1.));
#5598=CARTESIAN_POINT('Origin',(1.,0.,0.));
#6583=UNCERTAINTY_MEASURE_WITH_UNIT(LENGTH_MEASURE(0.001),#6639,
'DISTANCE_ACCURACY_VALUE',
'Maximum model space distance between geometric entities at asserted c
onnectivities');
#6609=UNCERTAINTY_MEASURE_WITH_UNIT(LENGTH_MEASURE(0.001),#6639,
'DISTANCE_ACCURACY_VALUE',
'Maximum model space distance between geometric entities at asserted c
onnectivities');
#6612=(
GEOMETRIC_REPRESENTATION_CONTEXT(3)
GLOBAL_UNCERTAINTY_ASSIGNED_CONTEXT((#6583))
GLOBAL_UNIT_ASSIGNED_CONTEXT((#6639,#6641,#6642))
REPRESENTATION_CONTEXT('','3D')
);
#6638=(
GEOMETRIC_REPRESENTATION_CONTEXT(3)
GLOBAL_UNCERTAINTY_ASSIGNED_CONTEXT((#6609))
GLOBAL_UNIT_ASSIGNED_CONTEXT((#6639,#6641,#6642))
REPRESENTATION_CONTEXT('','3D')
);
#6639=(
LENGTH_UNIT()
NAMED_UNIT(*)
SI_UNIT(.CENTI.,.METRE.)
);
#6641=(
NAMED_UNIT(*)
PLANE_ANGLE_UNIT()
SI_UNIT($,.RADIAN.)
);
#6642=(
NAMED_UNIT(*)
SI_UNIT($,.STERADIAN.)
SOLID_ANGLE_UNIT()
);
#6645=SHAPE_DEFINITION_REPRESENTATION(#6673,#6739);
#6673=PRODUCT_DEFINITION_SHAPE('',$,#6768);
#6739=SHAPE_REPRESENTATION('',(#3883),#6612);
#6765=PRODUCT_DEFINITION_CONTEXT('part definition',#6851,'design');
#6768=PRODUCT_DEFINITION('Base','Base',#6796,#6765);
#6796=PRODUCT_DEFINITION_FORMATION('',$,#6855);
#6851=APPLICATION_CONTEXT(
'Core Data for Automotive Mechanical Design Process');
#6852=PRODUCT_CONTEXT('part definition',#6851,'mechanical');
#6855=PRODUCT('Base','Base','Base',(#6852));
#6916=COLOUR_RGB('Dark Blue',0.08,0.2,0.34);
#6917=FILL_AREA_STYLE_COLOUR('',#6916);
#6918=FILL_AREA_STYLE('',(#6917));
#6919=SURFACE_STYLE_FILL_AREA(#6918);
#6920=SURFACE_SIDE_STYLE('',(#6919));
#6921=SURFACE_STYLE_USAGE(.BOTH.,#6920);
#6922=PRESENTATION_STYLE_ASSIGNMENT((#6921));
ENDSEC;
END-ISO-10303-21;
